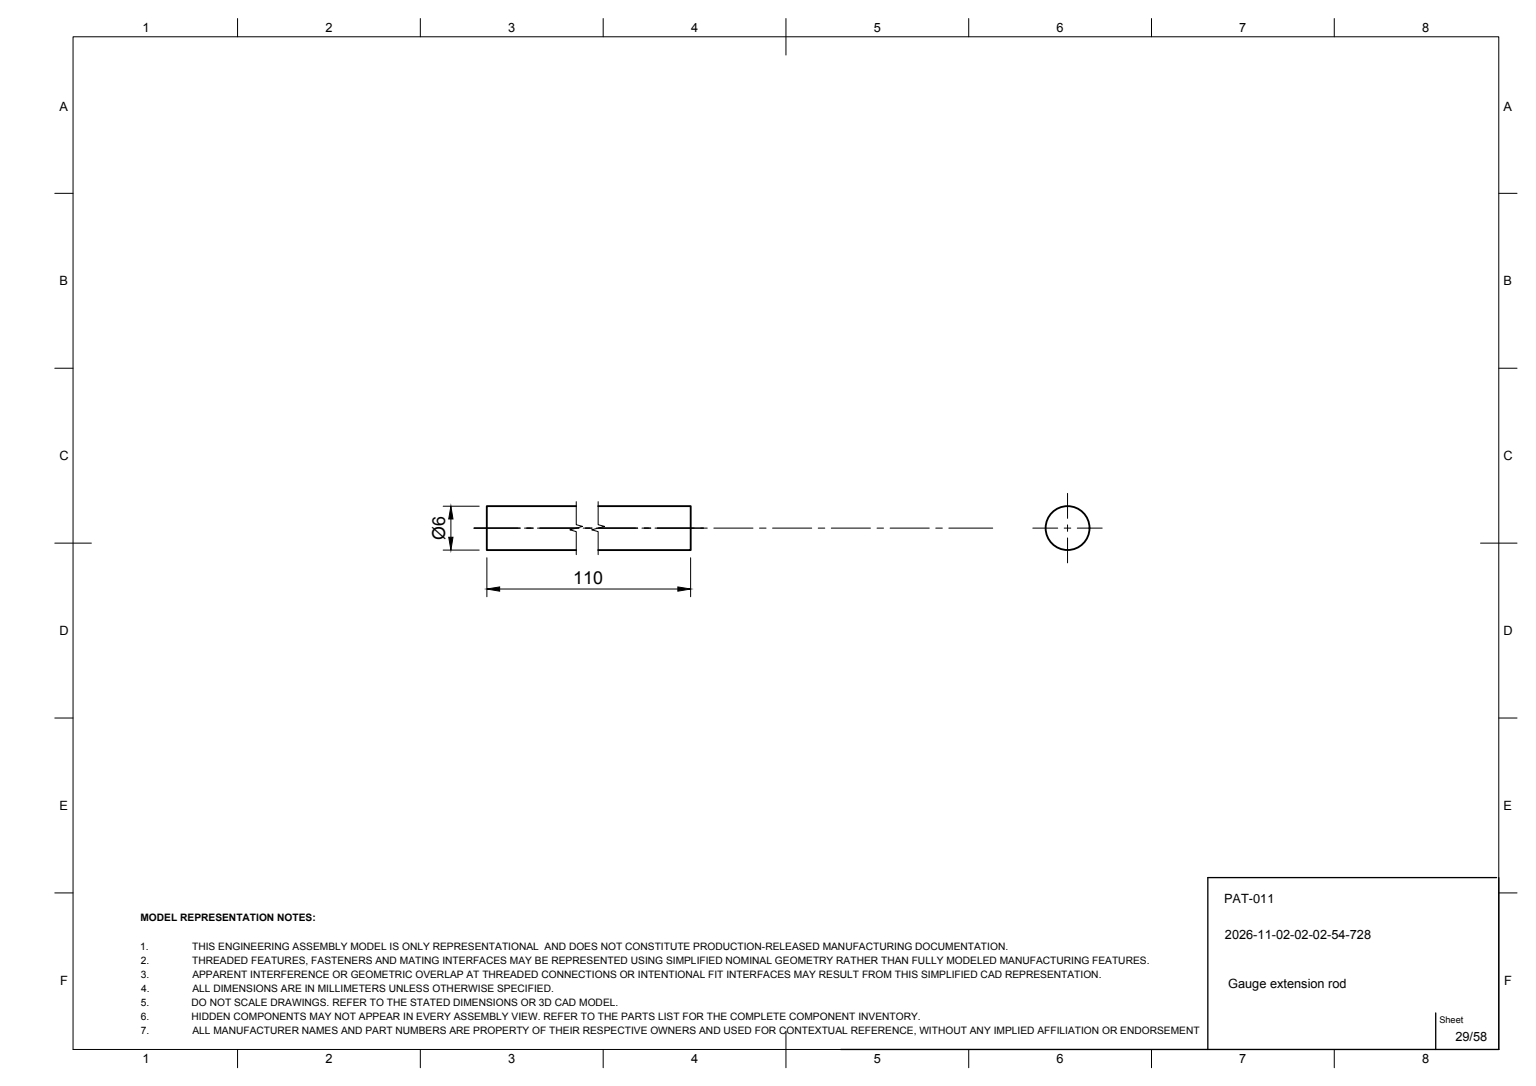
ISO-10303-21;
HEADER;
/* Generated by software containing ST-Developer
 * from STEP Tools, Inc. (www.steptools.com) 
 */

FILE_DESCRIPTION(
/* description */ ('Belt tension measurement rig'),
/* implementation_level */ '2;1');

FILE_NAME(
/* name */ 'Gauge extension rod.step',
/* time_stamp */ '2026-10-28T03:24:44-07:00',
/* author */ (''),
/* organization */ (''),
/* preprocessor_version */ 'ST-DEVELOPER v20.2',
/* originating_system */ 'Autodesk Translation Framework v15.17.0.0',
/* authorisation */ '');

FILE_SCHEMA (('AUTOMOTIVE_DESIGN { 1 0 10303 214 3 1 1 }'));
ENDSEC;

DATA;
#10=MECHANICAL_DESIGN_GEOMETRIC_PRESENTATION_REPRESENTATION('',(#725),#23587);
#607=SHAPE_REPRESENTATION_RELATIONSHIP('SRR','None',#23854,#662);
#662=ADVANCED_BREP_SHAPE_REPRESENTATION('',(#795),#23552);
#725=STYLED_ITEM('',(#24211),#795);
#795=MANIFOLD_SOLID_BREP('Body1',#12230);
#1191=PLANE('',#13543);
#1192=PLANE('',#13547);
#1664=FACE_OUTER_BOUND('',#2505,.T.);
#1665=FACE_OUTER_BOUND('',#2506,.T.);
#1666=FACE_OUTER_BOUND('',#2507,.T.);
#2505=EDGE_LOOP('',(#9304));
#2506=EDGE_LOOP('',(#9305,#9306,#9307,#9308));
#2507=EDGE_LOOP('',(#9309));
#3309=LINE('',#20457,#4060);
#4060=VECTOR('',#16198,0.3);
#4790=CIRCLE('',#13544,0.3);
#4791=CIRCLE('',#13546,0.3);
#5700=VERTEX_POINT('',#20453);
#5701=VERTEX_POINT('',#20456);
#7011=EDGE_CURVE('',#5700,#5700,#4790,.T.);
#7012=EDGE_CURVE('',#5700,#5701,#3309,.T.);
#7013=EDGE_CURVE('',#5701,#5701,#4791,.T.);
#9304=ORIENTED_EDGE('',*,*,#7011,.T.);
#9305=ORIENTED_EDGE('',*,*,#7011,.F.);
#9306=ORIENTED_EDGE('',*,*,#7012,.T.);
#9307=ORIENTED_EDGE('',*,*,#7013,.T.);
#9308=ORIENTED_EDGE('',*,*,#7012,.F.);
#9309=ORIENTED_EDGE('',*,*,#7013,.F.);
#11294=CYLINDRICAL_SURFACE('',#13545,0.3);
#11805=ADVANCED_FACE('',(#1664),#1191,.T.);
#11806=ADVANCED_FACE('',(#1665),#11294,.T.);
#11807=ADVANCED_FACE('',(#1666),#1192,.F.);
#12230=CLOSED_SHELL('',(#11805,#11806,#11807));
#13542=AXIS2_PLACEMENT_3D('',#20451,#16190,#16191);
#13543=AXIS2_PLACEMENT_3D('',#20452,#16192,#16193);
#13544=AXIS2_PLACEMENT_3D('',#20454,#16194,#16195);
#13545=AXIS2_PLACEMENT_3D('',#20455,#16196,#16197);
#13546=AXIS2_PLACEMENT_3D('',#20458,#16199,#16200);
#13547=AXIS2_PLACEMENT_3D('',#20459,#16201,#16202);
#16190=DIRECTION('axis',(0.,0.,1.));
#16191=DIRECTION('refdir',(1.,0.,0.));
#16192=DIRECTION('center_axis',(1.,0.,0.));
#16193=DIRECTION('ref_axis',(0.,0.,-1.));
#16194=DIRECTION('center_axis',(1.,0.,0.));
#16195=DIRECTION('ref_axis',(0.,0.,-1.));
#16196=DIRECTION('center_axis',(1.,0.,0.));
#16197=DIRECTION('ref_axis',(0.,0.,-1.));
#16198=DIRECTION('',(-1.,0.,0.));
#16199=DIRECTION('center_axis',(1.,0.,0.));
#16200=DIRECTION('ref_axis',(0.,0.,-1.));
#16201=DIRECTION('center_axis',(1.,0.,0.));
#16202=DIRECTION('ref_axis',(0.,0.,-1.));
#20451=CARTESIAN_POINT('',(0.,0.,0.));
#20452=CARTESIAN_POINT('Origin',(14.,7.5,4.5));
#20453=CARTESIAN_POINT('',(14.,7.5,4.8));
#20454=CARTESIAN_POINT('Origin',(14.,7.5,4.5));
#20455=CARTESIAN_POINT('Origin',(3.,7.5,4.5));
#20456=CARTESIAN_POINT('',(3.,7.5,4.8));
#20457=CARTESIAN_POINT('',(3.,7.5,4.8));
#20458=CARTESIAN_POINT('Origin',(3.,7.5,4.5));
#20459=CARTESIAN_POINT('Origin',(3.,7.5,4.5));
#23487=UNCERTAINTY_MEASURE_WITH_UNIT(LENGTH_MEASURE(0.001),#23588,
'DISTANCE_ACCURACY_VALUE',
'Maximum model space distance between geometric entities at asserted c
onnectivities');
#23522=UNCERTAINTY_MEASURE_WITH_UNIT(LENGTH_MEASURE(0.001),#23588,
'DISTANCE_ACCURACY_VALUE',
'Maximum model space distance between geometric entities at asserted c
onnectivities');
#23552=(
GEOMETRIC_REPRESENTATION_CONTEXT(3)
GLOBAL_UNCERTAINTY_ASSIGNED_CONTEXT((#23487))
GLOBAL_UNIT_ASSIGNED_CONTEXT((#23588,#23590,#23591))
REPRESENTATION_CONTEXT('','3D')
);
#23587=(
GEOMETRIC_REPRESENTATION_CONTEXT(3)
GLOBAL_UNCERTAINTY_ASSIGNED_CONTEXT((#23522))
GLOBAL_UNIT_ASSIGNED_CONTEXT((#23588,#23590,#23591))
REPRESENTATION_CONTEXT('','3D')
);
#23588=(
LENGTH_UNIT()
NAMED_UNIT(*)
SI_UNIT(.CENTI.,.METRE.)
);
#23590=(
NAMED_UNIT(*)
PLANE_ANGLE_UNIT()
SI_UNIT($,.RADIAN.)
);
#23591=(
NAMED_UNIT(*)
SI_UNIT($,.STERADIAN.)
SOLID_ANGLE_UNIT()
);
#23621=SHAPE_DEFINITION_REPRESENTATION(#23690,#23854);
#23690=PRODUCT_DEFINITION_SHAPE('',$,#23919);
#23854=SHAPE_REPRESENTATION('',(#13542),#23552);
#23889=PRODUCT_DEFINITION_CONTEXT('part definition',#24083,'design');
#23919=PRODUCT_DEFINITION('Gauge extension rod','Gauge extension rod',#23983,
#23889);
#23983=PRODUCT_DEFINITION_FORMATION('',$,#24114);
#24083=APPLICATION_CONTEXT(
'Core Data for Automotive Mechanical Design Process');
#24084=PRODUCT_CONTEXT('part definition',#24083,'mechanical');
#24114=PRODUCT('Gauge extension rod','Gauge extension rod',
'Gauge extension rod',(#24084));
#24205=COLOUR_RGB('Grey',0.48,0.52,0.57);
#24206=FILL_AREA_STYLE_COLOUR('',#24205);
#24207=FILL_AREA_STYLE('',(#24206));
#24208=SURFACE_STYLE_FILL_AREA(#24207);
#24209=SURFACE_SIDE_STYLE('',(#24208));
#24210=SURFACE_STYLE_USAGE(.BOTH.,#24209);
#24211=PRESENTATION_STYLE_ASSIGNMENT((#24210));
ENDSEC;
END-ISO-10303-21;
